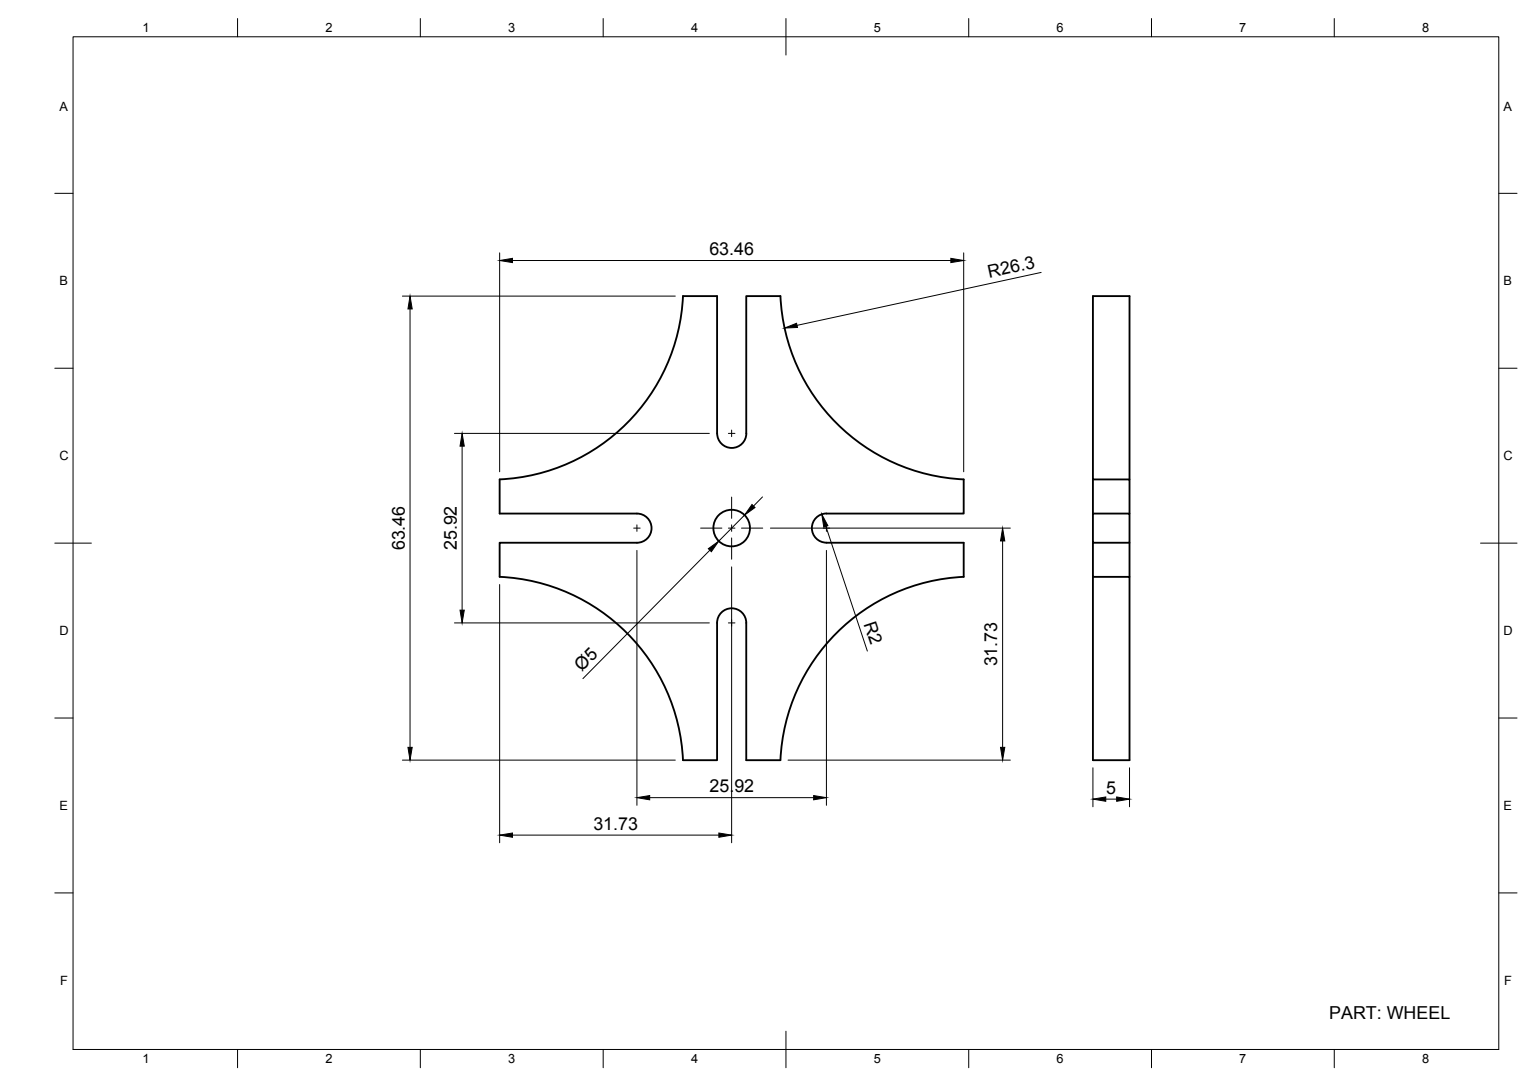
ISO-10303-21;
HEADER;
/* Generated by software containing ST-Developer
 * from STEP Tools, Inc. (www.steptools.com) 
 */

FILE_DESCRIPTION(
/* description */ (''),
/* implementation_level */ '2;1');

FILE_NAME(
/* name */ 'Wheel.step',
/* time_stamp */ '2026-09-20T21:52:48+06:00',
/* author */ (''),
/* organization */ (''),
/* preprocessor_version */ 'ST-DEVELOPER v20.2',
/* originating_system */ 'Autodesk Translation Framework v15.15.0.0',
/* authorisation */ '');

FILE_SCHEMA (('AUTOMOTIVE_DESIGN { 1 0 10303 214 3 1 1 }'));
ENDSEC;

DATA;
#10=MECHANICAL_DESIGN_GEOMETRIC_PRESENTATION_REPRESENTATION('',(#59),#2203);
#43=SHAPE_REPRESENTATION_RELATIONSHIP('SRR','None',#2235,#51);
#51=ADVANCED_BREP_SHAPE_REPRESENTATION('',(#67),#2195);
#59=STYLED_ITEM('',(#2284),#67);
#67=MANIFOLD_SOLID_BREP('Wheel',#1226);
#75=FACE_BOUND('',#256,.T.);
#76=FACE_BOUND('',#258,.T.);
#89=CIRCLE('',#1327,2.);
#90=CIRCLE('',#1328,2.);
#91=CIRCLE('',#1334,2.);
#92=CIRCLE('',#1335,2.);
#93=CIRCLE('',#1339,26.3);
#94=CIRCLE('',#1340,26.3);
#95=CIRCLE('',#1344,2.);
#96=CIRCLE('',#1345,2.);
#97=CIRCLE('',#1349,26.3);
#98=CIRCLE('',#1350,26.3);
#99=CIRCLE('',#1354,2.);
#100=CIRCLE('',#1355,2.);
#101=CIRCLE('',#1359,26.3);
#102=CIRCLE('',#1360,26.3);
#103=CIRCLE('',#1362,2.5);
#104=CIRCLE('',#1363,2.5);
#105=CIRCLE('',#1365,26.3);
#106=CIRCLE('',#1366,26.3);
#137=CYLINDRICAL_SURFACE('',#1326,2.);
#138=CYLINDRICAL_SURFACE('',#1333,2.);
#139=CYLINDRICAL_SURFACE('',#1338,26.3);
#140=CYLINDRICAL_SURFACE('',#1343,2.);
#141=CYLINDRICAL_SURFACE('',#1348,26.3);
#142=CYLINDRICAL_SURFACE('',#1353,2.);
#143=CYLINDRICAL_SURFACE('',#1358,26.3);
#144=CYLINDRICAL_SURFACE('',#1361,2.5);
#145=CYLINDRICAL_SURFACE('',#1364,26.3);
#161=FACE_OUTER_BOUND('',#230,.T.);
#162=FACE_OUTER_BOUND('',#231,.T.);
#163=FACE_OUTER_BOUND('',#232,.T.);
#164=FACE_OUTER_BOUND('',#233,.T.);
#165=FACE_OUTER_BOUND('',#234,.T.);
#166=FACE_OUTER_BOUND('',#235,.T.);
#167=FACE_OUTER_BOUND('',#236,.T.);
#168=FACE_OUTER_BOUND('',#237,.T.);
#169=FACE_OUTER_BOUND('',#238,.T.);
#170=FACE_OUTER_BOUND('',#239,.T.);
#171=FACE_OUTER_BOUND('',#240,.T.);
#172=FACE_OUTER_BOUND('',#241,.T.);
#173=FACE_OUTER_BOUND('',#242,.T.);
#174=FACE_OUTER_BOUND('',#243,.T.);
#175=FACE_OUTER_BOUND('',#244,.T.);
#176=FACE_OUTER_BOUND('',#245,.T.);
#177=FACE_OUTER_BOUND('',#246,.T.);
#178=FACE_OUTER_BOUND('',#247,.T.);
#179=FACE_OUTER_BOUND('',#248,.T.);
#180=FACE_OUTER_BOUND('',#249,.T.);
#181=FACE_OUTER_BOUND('',#250,.T.);
#182=FACE_OUTER_BOUND('',#251,.T.);
#183=FACE_OUTER_BOUND('',#252,.T.);
#184=FACE_OUTER_BOUND('',#253,.T.);
#185=FACE_OUTER_BOUND('',#254,.T.);
#186=FACE_OUTER_BOUND('',#255,.T.);
#187=FACE_OUTER_BOUND('',#257,.T.);
#230=EDGE_LOOP('',(#796,#797,#798,#799));
#231=EDGE_LOOP('',(#800,#801,#802,#803));
#232=EDGE_LOOP('',(#804,#805,#806,#807));
#233=EDGE_LOOP('',(#808,#809,#810,#811));
#234=EDGE_LOOP('',(#812,#813,#814,#815));
#235=EDGE_LOOP('',(#816,#817,#818,#819));
#236=EDGE_LOOP('',(#820,#821,#822,#823));
#237=EDGE_LOOP('',(#824,#825,#826,#827));
#238=EDGE_LOOP('',(#828,#829,#830,#831));
#239=EDGE_LOOP('',(#832,#833,#834,#835));
#240=EDGE_LOOP('',(#836,#837,#838,#839));
#241=EDGE_LOOP('',(#840,#841,#842,#843));
#242=EDGE_LOOP('',(#844,#845,#846,#847));
#243=EDGE_LOOP('',(#848,#849,#850,#851));
#244=EDGE_LOOP('',(#852,#853,#854,#855));
#245=EDGE_LOOP('',(#856,#857,#858,#859));
#246=EDGE_LOOP('',(#860,#861,#862,#863));
#247=EDGE_LOOP('',(#864,#865,#866,#867));
#248=EDGE_LOOP('',(#868,#869,#870,#871));
#249=EDGE_LOOP('',(#872,#873,#874,#875));
#250=EDGE_LOOP('',(#876,#877,#878,#879));
#251=EDGE_LOOP('',(#880,#881,#882,#883));
#252=EDGE_LOOP('',(#884,#885,#886,#887));
#253=EDGE_LOOP('',(#888,#889,#890,#891));
#254=EDGE_LOOP('',(#892,#893,#894,#895));
#255=EDGE_LOOP('',(#896,#897,#898,#899,#900,#901,#902,#903,#904,#905,#906,
#907,#908,#909,#910,#911,#912,#913,#914,#915,#916,#917,#918,#919));
#256=EDGE_LOOP('',(#920));
#257=EDGE_LOOP('',(#921,#922,#923,#924,#925,#926,#927,#928,#929,#930,#931,
#932,#933,#934,#935,#936,#937,#938,#939,#940,#941,#942,#943,#944));
#258=EDGE_LOOP('',(#945));
#313=LINE('',#1840,#423);
#314=LINE('',#1842,#424);
#315=LINE('',#1844,#425);
#316=LINE('',#1845,#426);
#317=LINE('',#1851,#427);
#318=LINE('',#1854,#428);
#319=LINE('',#1856,#429);
#320=LINE('',#1857,#430);
#321=LINE('',#1860,#431);
#322=LINE('',#1862,#432);
#323=LINE('',#1863,#433);
#324=LINE('',#1866,#434);
#325=LINE('',#1868,#435);
#326=LINE('',#1869,#436);
#327=LINE('',#1873,#437);
#328=LINE('',#1875,#438);
#329=LINE('',#1877,#439);
#330=LINE('',#1878,#440);
#331=LINE('',#1883,#441);
#332=LINE('',#1887,#442);
#333=LINE('',#1889,#443);
#334=LINE('',#1890,#444);
#335=LINE('',#1893,#445);
#336=LINE('',#1895,#446);
#337=LINE('',#1896,#447);
#338=LINE('',#1902,#448);
#339=LINE('',#1904,#449);
#340=LINE('',#1905,#450);
#341=LINE('',#1909,#451);
#342=LINE('',#1911,#452);
#343=LINE('',#1913,#453);
#344=LINE('',#1914,#454);
#345=LINE('',#1919,#455);
#346=LINE('',#1923,#456);
#347=LINE('',#1925,#457);
#348=LINE('',#1926,#458);
#349=LINE('',#1929,#459);
#350=LINE('',#1931,#460);
#351=LINE('',#1932,#461);
#352=LINE('',#1937,#462);
#353=LINE('',#1940,#463);
#354=LINE('',#1941,#464);
#355=LINE('',#1945,#465);
#356=LINE('',#1947,#466);
#357=LINE('',#1949,#467);
#358=LINE('',#1950,#468);
#359=LINE('',#1956,#469);
#360=LINE('',#1959,#470);
#361=LINE('',#1961,#471);
#362=LINE('',#1962,#472);
#363=LINE('',#1965,#473);
#364=LINE('',#1967,#474);
#365=LINE('',#1968,#475);
#366=LINE('',#1976,#476);
#367=LINE('',#1983,#477);
#368=LINE('',#1985,#478);
#369=LINE('',#1986,#479);
#423=VECTOR('',#1463,10.);
#424=VECTOR('',#1464,10.);
#425=VECTOR('',#1465,10.);
#426=VECTOR('',#1466,10.);
#427=VECTOR('',#1473,10.);
#428=VECTOR('',#1476,10.);
#429=VECTOR('',#1477,10.);
#430=VECTOR('',#1478,10.);
#431=VECTOR('',#1481,10.);
#432=VECTOR('',#1482,10.);
#433=VECTOR('',#1483,10.);
#434=VECTOR('',#1486,10.);
#435=VECTOR('',#1487,10.);
#436=VECTOR('',#1488,10.);
#437=VECTOR('',#1491,10.);
#438=VECTOR('',#1492,10.);
#439=VECTOR('',#1493,10.);
#440=VECTOR('',#1494,10.);
#441=VECTOR('',#1499,10.);
#442=VECTOR('',#1504,10.);
#443=VECTOR('',#1505,10.);
#444=VECTOR('',#1506,10.);
#445=VECTOR('',#1509,10.);
#446=VECTOR('',#1510,10.);
#447=VECTOR('',#1511,10.);
#448=VECTOR('',#1520,10.);
#449=VECTOR('',#1521,10.);
#450=VECTOR('',#1522,10.);
#451=VECTOR('',#1525,10.);
#452=VECTOR('',#1526,10.);
#453=VECTOR('',#1527,10.);
#454=VECTOR('',#1528,10.);
#455=VECTOR('',#1533,10.);
#456=VECTOR('',#1538,10.);
#457=VECTOR('',#1539,10.);
#458=VECTOR('',#1540,10.);
#459=VECTOR('',#1543,10.);
#460=VECTOR('',#1544,10.);
#461=VECTOR('',#1545,10.);
#462=VECTOR('',#1550,10.);
#463=VECTOR('',#1555,10.);
#464=VECTOR('',#1556,10.);
#465=VECTOR('',#1559,10.);
#466=VECTOR('',#1560,10.);
#467=VECTOR('',#1561,10.);
#468=VECTOR('',#1562,10.);
#469=VECTOR('',#1569,10.);
#470=VECTOR('',#1572,10.);
#471=VECTOR('',#1573,10.);
#472=VECTOR('',#1574,10.);
#473=VECTOR('',#1577,10.);
#474=VECTOR('',#1578,10.);
#475=VECTOR('',#1579,10.);
#476=VECTOR('',#1590,2.5);
#477=VECTOR('',#1599,10.);
#478=VECTOR('',#1602,10.);
#479=VECTOR('',#1603,10.);
#533=VERTEX_POINT('',#1838);
#534=VERTEX_POINT('',#1839);
#535=VERTEX_POINT('',#1841);
#536=VERTEX_POINT('',#1843);
#537=VERTEX_POINT('',#1847);
#538=VERTEX_POINT('',#1849);
#539=VERTEX_POINT('',#1853);
#540=VERTEX_POINT('',#1855);
#541=VERTEX_POINT('',#1859);
#542=VERTEX_POINT('',#1861);
#543=VERTEX_POINT('',#1865);
#544=VERTEX_POINT('',#1867);
#545=VERTEX_POINT('',#1871);
#546=VERTEX_POINT('',#1872);
#547=VERTEX_POINT('',#1874);
#548=VERTEX_POINT('',#1876);
#549=VERTEX_POINT('',#1880);
#550=VERTEX_POINT('',#1882);
#551=VERTEX_POINT('',#1886);
#552=VERTEX_POINT('',#1888);
#553=VERTEX_POINT('',#1892);
#554=VERTEX_POINT('',#1894);
#555=VERTEX_POINT('',#1901);
#556=VERTEX_POINT('',#1903);
#557=VERTEX_POINT('',#1907);
#558=VERTEX_POINT('',#1908);
#559=VERTEX_POINT('',#1910);
#560=VERTEX_POINT('',#1912);
#561=VERTEX_POINT('',#1916);
#562=VERTEX_POINT('',#1918);
#563=VERTEX_POINT('',#1922);
#564=VERTEX_POINT('',#1924);
#565=VERTEX_POINT('',#1928);
#566=VERTEX_POINT('',#1930);
#567=VERTEX_POINT('',#1934);
#568=VERTEX_POINT('',#1936);
#569=VERTEX_POINT('',#1943);
#570=VERTEX_POINT('',#1944);
#571=VERTEX_POINT('',#1946);
#572=VERTEX_POINT('',#1948);
#573=VERTEX_POINT('',#1952);
#574=VERTEX_POINT('',#1954);
#575=VERTEX_POINT('',#1958);
#576=VERTEX_POINT('',#1960);
#577=VERTEX_POINT('',#1964);
#578=VERTEX_POINT('',#1966);
#579=VERTEX_POINT('',#1973);
#580=VERTEX_POINT('',#1975);
#581=VERTEX_POINT('',#1979);
#582=VERTEX_POINT('',#1981);
#638=EDGE_CURVE('',#533,#534,#313,.T.);
#639=EDGE_CURVE('',#534,#535,#314,.T.);
#640=EDGE_CURVE('',#536,#535,#315,.T.);
#641=EDGE_CURVE('',#533,#536,#316,.T.);
#642=EDGE_CURVE('',#537,#533,#89,.T.);
#643=EDGE_CURVE('',#538,#536,#90,.T.);
#644=EDGE_CURVE('',#537,#538,#317,.T.);
#645=EDGE_CURVE('',#539,#537,#318,.T.);
#646=EDGE_CURVE('',#540,#538,#319,.T.);
#647=EDGE_CURVE('',#539,#540,#320,.T.);
#648=EDGE_CURVE('',#539,#541,#321,.T.);
#649=EDGE_CURVE('',#542,#540,#322,.T.);
#650=EDGE_CURVE('',#541,#542,#323,.T.);
#651=EDGE_CURVE('',#543,#534,#324,.T.);
#652=EDGE_CURVE('',#543,#544,#325,.T.);
#653=EDGE_CURVE('',#535,#544,#326,.T.);
#654=EDGE_CURVE('',#545,#546,#327,.T.);
#655=EDGE_CURVE('',#545,#547,#328,.T.);
#656=EDGE_CURVE('',#547,#548,#329,.T.);
#657=EDGE_CURVE('',#546,#548,#330,.T.);
#658=EDGE_CURVE('',#549,#545,#91,.T.);
#659=EDGE_CURVE('',#549,#550,#331,.T.);
#660=EDGE_CURVE('',#550,#547,#92,.T.);
#661=EDGE_CURVE('',#551,#549,#332,.T.);
#662=EDGE_CURVE('',#551,#552,#333,.T.);
#663=EDGE_CURVE('',#552,#550,#334,.T.);
#664=EDGE_CURVE('',#551,#553,#335,.T.);
#665=EDGE_CURVE('',#553,#554,#336,.T.);
#666=EDGE_CURVE('',#554,#552,#337,.T.);
#667=EDGE_CURVE('',#541,#553,#93,.T.);
#668=EDGE_CURVE('',#554,#542,#94,.T.);
#669=EDGE_CURVE('',#555,#546,#338,.T.);
#670=EDGE_CURVE('',#548,#556,#339,.T.);
#671=EDGE_CURVE('',#555,#556,#340,.T.);
#672=EDGE_CURVE('',#557,#558,#341,.T.);
#673=EDGE_CURVE('',#557,#559,#342,.T.);
#674=EDGE_CURVE('',#559,#560,#343,.T.);
#675=EDGE_CURVE('',#558,#560,#344,.T.);
#676=EDGE_CURVE('',#561,#557,#95,.T.);
#677=EDGE_CURVE('',#561,#562,#345,.T.);
#678=EDGE_CURVE('',#562,#559,#96,.T.);
#679=EDGE_CURVE('',#563,#561,#346,.T.);
#680=EDGE_CURVE('',#563,#564,#347,.T.);
#681=EDGE_CURVE('',#564,#562,#348,.T.);
#682=EDGE_CURVE('',#563,#565,#349,.T.);
#683=EDGE_CURVE('',#565,#566,#350,.T.);
#684=EDGE_CURVE('',#566,#564,#351,.T.);
#685=EDGE_CURVE('',#543,#567,#97,.T.);
#686=EDGE_CURVE('',#567,#568,#352,.T.);
#687=EDGE_CURVE('',#544,#568,#98,.T.);
#688=EDGE_CURVE('',#567,#558,#353,.T.);
#689=EDGE_CURVE('',#560,#568,#354,.T.);
#690=EDGE_CURVE('',#569,#570,#355,.T.);
#691=EDGE_CURVE('',#570,#571,#356,.T.);
#692=EDGE_CURVE('',#572,#571,#357,.T.);
#693=EDGE_CURVE('',#569,#572,#358,.T.);
#694=EDGE_CURVE('',#573,#569,#99,.T.);
#695=EDGE_CURVE('',#574,#572,#100,.T.);
#696=EDGE_CURVE('',#573,#574,#359,.T.);
#697=EDGE_CURVE('',#575,#573,#360,.T.);
#698=EDGE_CURVE('',#576,#574,#361,.T.);
#699=EDGE_CURVE('',#575,#576,#362,.T.);
#700=EDGE_CURVE('',#575,#577,#363,.T.);
#701=EDGE_CURVE('',#578,#576,#364,.T.);
#702=EDGE_CURVE('',#577,#578,#365,.T.);
#703=EDGE_CURVE('',#565,#577,#101,.T.);
#704=EDGE_CURVE('',#578,#566,#102,.T.);
#705=EDGE_CURVE('',#579,#579,#103,.T.);
#706=EDGE_CURVE('',#579,#580,#366,.T.);
#707=EDGE_CURVE('',#580,#580,#104,.T.);
#708=EDGE_CURVE('',#581,#555,#105,.T.);
#709=EDGE_CURVE('',#582,#556,#106,.T.);
#710=EDGE_CURVE('',#581,#582,#367,.T.);
#711=EDGE_CURVE('',#581,#570,#368,.T.);
#712=EDGE_CURVE('',#571,#582,#369,.T.);
#796=ORIENTED_EDGE('',*,*,#638,.T.);
#797=ORIENTED_EDGE('',*,*,#639,.T.);
#798=ORIENTED_EDGE('',*,*,#640,.F.);
#799=ORIENTED_EDGE('',*,*,#641,.F.);
#800=ORIENTED_EDGE('',*,*,#642,.T.);
#801=ORIENTED_EDGE('',*,*,#641,.T.);
#802=ORIENTED_EDGE('',*,*,#643,.F.);
#803=ORIENTED_EDGE('',*,*,#644,.F.);
#804=ORIENTED_EDGE('',*,*,#645,.T.);
#805=ORIENTED_EDGE('',*,*,#644,.T.);
#806=ORIENTED_EDGE('',*,*,#646,.F.);
#807=ORIENTED_EDGE('',*,*,#647,.F.);
#808=ORIENTED_EDGE('',*,*,#648,.F.);
#809=ORIENTED_EDGE('',*,*,#647,.T.);
#810=ORIENTED_EDGE('',*,*,#649,.F.);
#811=ORIENTED_EDGE('',*,*,#650,.F.);
#812=ORIENTED_EDGE('',*,*,#651,.F.);
#813=ORIENTED_EDGE('',*,*,#652,.T.);
#814=ORIENTED_EDGE('',*,*,#653,.F.);
#815=ORIENTED_EDGE('',*,*,#639,.F.);
#816=ORIENTED_EDGE('',*,*,#654,.F.);
#817=ORIENTED_EDGE('',*,*,#655,.T.);
#818=ORIENTED_EDGE('',*,*,#656,.T.);
#819=ORIENTED_EDGE('',*,*,#657,.F.);
#820=ORIENTED_EDGE('',*,*,#658,.F.);
#821=ORIENTED_EDGE('',*,*,#659,.T.);
#822=ORIENTED_EDGE('',*,*,#660,.T.);
#823=ORIENTED_EDGE('',*,*,#655,.F.);
#824=ORIENTED_EDGE('',*,*,#661,.F.);
#825=ORIENTED_EDGE('',*,*,#662,.T.);
#826=ORIENTED_EDGE('',*,*,#663,.T.);
#827=ORIENTED_EDGE('',*,*,#659,.F.);
#828=ORIENTED_EDGE('',*,*,#664,.T.);
#829=ORIENTED_EDGE('',*,*,#665,.T.);
#830=ORIENTED_EDGE('',*,*,#666,.T.);
#831=ORIENTED_EDGE('',*,*,#662,.F.);
#832=ORIENTED_EDGE('',*,*,#667,.F.);
#833=ORIENTED_EDGE('',*,*,#650,.T.);
#834=ORIENTED_EDGE('',*,*,#668,.F.);
#835=ORIENTED_EDGE('',*,*,#665,.F.);
#836=ORIENTED_EDGE('',*,*,#669,.T.);
#837=ORIENTED_EDGE('',*,*,#657,.T.);
#838=ORIENTED_EDGE('',*,*,#670,.T.);
#839=ORIENTED_EDGE('',*,*,#671,.F.);
#840=ORIENTED_EDGE('',*,*,#672,.F.);
#841=ORIENTED_EDGE('',*,*,#673,.T.);
#842=ORIENTED_EDGE('',*,*,#674,.T.);
#843=ORIENTED_EDGE('',*,*,#675,.F.);
#844=ORIENTED_EDGE('',*,*,#676,.F.);
#845=ORIENTED_EDGE('',*,*,#677,.T.);
#846=ORIENTED_EDGE('',*,*,#678,.T.);
#847=ORIENTED_EDGE('',*,*,#673,.F.);
#848=ORIENTED_EDGE('',*,*,#679,.F.);
#849=ORIENTED_EDGE('',*,*,#680,.T.);
#850=ORIENTED_EDGE('',*,*,#681,.T.);
#851=ORIENTED_EDGE('',*,*,#677,.F.);
#852=ORIENTED_EDGE('',*,*,#682,.T.);
#853=ORIENTED_EDGE('',*,*,#683,.T.);
#854=ORIENTED_EDGE('',*,*,#684,.T.);
#855=ORIENTED_EDGE('',*,*,#680,.F.);
#856=ORIENTED_EDGE('',*,*,#685,.T.);
#857=ORIENTED_EDGE('',*,*,#686,.T.);
#858=ORIENTED_EDGE('',*,*,#687,.F.);
#859=ORIENTED_EDGE('',*,*,#652,.F.);
#860=ORIENTED_EDGE('',*,*,#688,.T.);
#861=ORIENTED_EDGE('',*,*,#675,.T.);
#862=ORIENTED_EDGE('',*,*,#689,.T.);
#863=ORIENTED_EDGE('',*,*,#686,.F.);
#864=ORIENTED_EDGE('',*,*,#690,.T.);
#865=ORIENTED_EDGE('',*,*,#691,.T.);
#866=ORIENTED_EDGE('',*,*,#692,.F.);
#867=ORIENTED_EDGE('',*,*,#693,.F.);
#868=ORIENTED_EDGE('',*,*,#694,.T.);
#869=ORIENTED_EDGE('',*,*,#693,.T.);
#870=ORIENTED_EDGE('',*,*,#695,.F.);
#871=ORIENTED_EDGE('',*,*,#696,.F.);
#872=ORIENTED_EDGE('',*,*,#697,.T.);
#873=ORIENTED_EDGE('',*,*,#696,.T.);
#874=ORIENTED_EDGE('',*,*,#698,.F.);
#875=ORIENTED_EDGE('',*,*,#699,.F.);
#876=ORIENTED_EDGE('',*,*,#700,.F.);
#877=ORIENTED_EDGE('',*,*,#699,.T.);
#878=ORIENTED_EDGE('',*,*,#701,.F.);
#879=ORIENTED_EDGE('',*,*,#702,.F.);
#880=ORIENTED_EDGE('',*,*,#703,.T.);
#881=ORIENTED_EDGE('',*,*,#702,.T.);
#882=ORIENTED_EDGE('',*,*,#704,.T.);
#883=ORIENTED_EDGE('',*,*,#683,.F.);
#884=ORIENTED_EDGE('',*,*,#705,.T.);
#885=ORIENTED_EDGE('',*,*,#706,.T.);
#886=ORIENTED_EDGE('',*,*,#707,.T.);
#887=ORIENTED_EDGE('',*,*,#706,.F.);
#888=ORIENTED_EDGE('',*,*,#708,.T.);
#889=ORIENTED_EDGE('',*,*,#671,.T.);
#890=ORIENTED_EDGE('',*,*,#709,.F.);
#891=ORIENTED_EDGE('',*,*,#710,.F.);
#892=ORIENTED_EDGE('',*,*,#711,.F.);
#893=ORIENTED_EDGE('',*,*,#710,.T.);
#894=ORIENTED_EDGE('',*,*,#712,.F.);
#895=ORIENTED_EDGE('',*,*,#691,.F.);
#896=ORIENTED_EDGE('',*,*,#685,.F.);
#897=ORIENTED_EDGE('',*,*,#651,.T.);
#898=ORIENTED_EDGE('',*,*,#638,.F.);
#899=ORIENTED_EDGE('',*,*,#642,.F.);
#900=ORIENTED_EDGE('',*,*,#645,.F.);
#901=ORIENTED_EDGE('',*,*,#648,.T.);
#902=ORIENTED_EDGE('',*,*,#667,.T.);
#903=ORIENTED_EDGE('',*,*,#664,.F.);
#904=ORIENTED_EDGE('',*,*,#661,.T.);
#905=ORIENTED_EDGE('',*,*,#658,.T.);
#906=ORIENTED_EDGE('',*,*,#654,.T.);
#907=ORIENTED_EDGE('',*,*,#669,.F.);
#908=ORIENTED_EDGE('',*,*,#708,.F.);
#909=ORIENTED_EDGE('',*,*,#711,.T.);
#910=ORIENTED_EDGE('',*,*,#690,.F.);
#911=ORIENTED_EDGE('',*,*,#694,.F.);
#912=ORIENTED_EDGE('',*,*,#697,.F.);
#913=ORIENTED_EDGE('',*,*,#700,.T.);
#914=ORIENTED_EDGE('',*,*,#703,.F.);
#915=ORIENTED_EDGE('',*,*,#682,.F.);
#916=ORIENTED_EDGE('',*,*,#679,.T.);
#917=ORIENTED_EDGE('',*,*,#676,.T.);
#918=ORIENTED_EDGE('',*,*,#672,.T.);
#919=ORIENTED_EDGE('',*,*,#688,.F.);
#920=ORIENTED_EDGE('',*,*,#707,.F.);
#921=ORIENTED_EDGE('',*,*,#687,.T.);
#922=ORIENTED_EDGE('',*,*,#689,.F.);
#923=ORIENTED_EDGE('',*,*,#674,.F.);
#924=ORIENTED_EDGE('',*,*,#678,.F.);
#925=ORIENTED_EDGE('',*,*,#681,.F.);
#926=ORIENTED_EDGE('',*,*,#684,.F.);
#927=ORIENTED_EDGE('',*,*,#704,.F.);
#928=ORIENTED_EDGE('',*,*,#701,.T.);
#929=ORIENTED_EDGE('',*,*,#698,.T.);
#930=ORIENTED_EDGE('',*,*,#695,.T.);
#931=ORIENTED_EDGE('',*,*,#692,.T.);
#932=ORIENTED_EDGE('',*,*,#712,.T.);
#933=ORIENTED_EDGE('',*,*,#709,.T.);
#934=ORIENTED_EDGE('',*,*,#670,.F.);
#935=ORIENTED_EDGE('',*,*,#656,.F.);
#936=ORIENTED_EDGE('',*,*,#660,.F.);
#937=ORIENTED_EDGE('',*,*,#663,.F.);
#938=ORIENTED_EDGE('',*,*,#666,.F.);
#939=ORIENTED_EDGE('',*,*,#668,.T.);
#940=ORIENTED_EDGE('',*,*,#649,.T.);
#941=ORIENTED_EDGE('',*,*,#646,.T.);
#942=ORIENTED_EDGE('',*,*,#643,.T.);
#943=ORIENTED_EDGE('',*,*,#640,.T.);
#944=ORIENTED_EDGE('',*,*,#653,.T.);
#945=ORIENTED_EDGE('',*,*,#705,.F.);
#1112=PLANE('',#1325);
#1113=PLANE('',#1329);
#1114=PLANE('',#1330);
#1115=PLANE('',#1331);
#1116=PLANE('',#1332);
#1117=PLANE('',#1336);
#1118=PLANE('',#1337);
#1119=PLANE('',#1341);
#1120=PLANE('',#1342);
#1121=PLANE('',#1346);
#1122=PLANE('',#1347);
#1123=PLANE('',#1351);
#1124=PLANE('',#1352);
#1125=PLANE('',#1356);
#1126=PLANE('',#1357);
#1127=PLANE('',#1367);
#1128=PLANE('',#1368);
#1129=PLANE('',#1369);
#1157=ADVANCED_FACE('',(#161),#1112,.T.);
#1158=ADVANCED_FACE('',(#162),#137,.F.);
#1159=ADVANCED_FACE('',(#163),#1113,.T.);
#1160=ADVANCED_FACE('',(#164),#1114,.T.);
#1161=ADVANCED_FACE('',(#165),#1115,.T.);
#1162=ADVANCED_FACE('',(#166),#1116,.F.);
#1163=ADVANCED_FACE('',(#167),#138,.F.);
#1164=ADVANCED_FACE('',(#168),#1117,.F.);
#1165=ADVANCED_FACE('',(#169),#1118,.F.);
#1166=ADVANCED_FACE('',(#170),#139,.F.);
#1167=ADVANCED_FACE('',(#171),#1119,.F.);
#1168=ADVANCED_FACE('',(#172),#1120,.F.);
#1169=ADVANCED_FACE('',(#173),#140,.F.);
#1170=ADVANCED_FACE('',(#174),#1121,.F.);
#1171=ADVANCED_FACE('',(#175),#1122,.F.);
#1172=ADVANCED_FACE('',(#176),#141,.F.);
#1173=ADVANCED_FACE('',(#177),#1123,.F.);
#1174=ADVANCED_FACE('',(#178),#1124,.T.);
#1175=ADVANCED_FACE('',(#179),#142,.F.);
#1176=ADVANCED_FACE('',(#180),#1125,.T.);
#1177=ADVANCED_FACE('',(#181),#1126,.T.);
#1178=ADVANCED_FACE('',(#182),#143,.F.);
#1179=ADVANCED_FACE('',(#183),#144,.F.);
#1180=ADVANCED_FACE('',(#184),#145,.F.);
#1181=ADVANCED_FACE('',(#185),#1127,.T.);
#1182=ADVANCED_FACE('',(#186,#75),#1128,.T.);
#1183=ADVANCED_FACE('',(#187,#76),#1129,.F.);
#1226=CLOSED_SHELL('',(#1157,#1158,#1159,#1160,#1161,#1162,#1163,#1164,
#1165,#1166,#1167,#1168,#1169,#1170,#1171,#1172,#1173,#1174,#1175,#1176,
#1177,#1178,#1179,#1180,#1181,#1182,#1183));
#1324=AXIS2_PLACEMENT_3D('',#1836,#1459,#1460);
#1325=AXIS2_PLACEMENT_3D('',#1837,#1461,#1462);
#1326=AXIS2_PLACEMENT_3D('',#1846,#1467,#1468);
#1327=AXIS2_PLACEMENT_3D('',#1848,#1469,#1470);
#1328=AXIS2_PLACEMENT_3D('',#1850,#1471,#1472);
#1329=AXIS2_PLACEMENT_3D('',#1852,#1474,#1475);
#1330=AXIS2_PLACEMENT_3D('',#1858,#1479,#1480);
#1331=AXIS2_PLACEMENT_3D('',#1864,#1484,#1485);
#1332=AXIS2_PLACEMENT_3D('',#1870,#1489,#1490);
#1333=AXIS2_PLACEMENT_3D('',#1879,#1495,#1496);
#1334=AXIS2_PLACEMENT_3D('',#1881,#1497,#1498);
#1335=AXIS2_PLACEMENT_3D('',#1884,#1500,#1501);
#1336=AXIS2_PLACEMENT_3D('',#1885,#1502,#1503);
#1337=AXIS2_PLACEMENT_3D('',#1891,#1507,#1508);
#1338=AXIS2_PLACEMENT_3D('',#1897,#1512,#1513);
#1339=AXIS2_PLACEMENT_3D('',#1898,#1514,#1515);
#1340=AXIS2_PLACEMENT_3D('',#1899,#1516,#1517);
#1341=AXIS2_PLACEMENT_3D('',#1900,#1518,#1519);
#1342=AXIS2_PLACEMENT_3D('',#1906,#1523,#1524);
#1343=AXIS2_PLACEMENT_3D('',#1915,#1529,#1530);
#1344=AXIS2_PLACEMENT_3D('',#1917,#1531,#1532);
#1345=AXIS2_PLACEMENT_3D('',#1920,#1534,#1535);
#1346=AXIS2_PLACEMENT_3D('',#1921,#1536,#1537);
#1347=AXIS2_PLACEMENT_3D('',#1927,#1541,#1542);
#1348=AXIS2_PLACEMENT_3D('',#1933,#1546,#1547);
#1349=AXIS2_PLACEMENT_3D('',#1935,#1548,#1549);
#1350=AXIS2_PLACEMENT_3D('',#1938,#1551,#1552);
#1351=AXIS2_PLACEMENT_3D('',#1939,#1553,#1554);
#1352=AXIS2_PLACEMENT_3D('',#1942,#1557,#1558);
#1353=AXIS2_PLACEMENT_3D('',#1951,#1563,#1564);
#1354=AXIS2_PLACEMENT_3D('',#1953,#1565,#1566);
#1355=AXIS2_PLACEMENT_3D('',#1955,#1567,#1568);
#1356=AXIS2_PLACEMENT_3D('',#1957,#1570,#1571);
#1357=AXIS2_PLACEMENT_3D('',#1963,#1575,#1576);
#1358=AXIS2_PLACEMENT_3D('',#1969,#1580,#1581);
#1359=AXIS2_PLACEMENT_3D('',#1970,#1582,#1583);
#1360=AXIS2_PLACEMENT_3D('',#1971,#1584,#1585);
#1361=AXIS2_PLACEMENT_3D('',#1972,#1586,#1587);
#1362=AXIS2_PLACEMENT_3D('',#1974,#1588,#1589);
#1363=AXIS2_PLACEMENT_3D('',#1977,#1591,#1592);
#1364=AXIS2_PLACEMENT_3D('',#1978,#1593,#1594);
#1365=AXIS2_PLACEMENT_3D('',#1980,#1595,#1596);
#1366=AXIS2_PLACEMENT_3D('',#1982,#1597,#1598);
#1367=AXIS2_PLACEMENT_3D('',#1984,#1600,#1601);
#1368=AXIS2_PLACEMENT_3D('',#1987,#1604,#1605);
#1369=AXIS2_PLACEMENT_3D('',#1988,#1606,#1607);
#1459=DIRECTION('axis',(0.,0.,1.));
#1460=DIRECTION('refdir',(1.,0.,0.));
#1461=DIRECTION('center_axis',(0.707106781186548,0.,-0.707106781186547));
#1462=DIRECTION('ref_axis',(0.707106781186547,0.,0.707106781186548));
#1463=DIRECTION('',(0.707106781186547,0.,0.707106781186548));
#1464=DIRECTION('',(0.,-1.,0.));
#1465=DIRECTION('',(0.707106781186547,0.,0.707106781186548));
#1466=DIRECTION('',(0.,-1.,0.));
#1467=DIRECTION('center_axis',(0.,-1.,0.));
#1468=DIRECTION('ref_axis',(0.707106781186549,0.,-0.707106781186546));
#1469=DIRECTION('center_axis',(0.,1.,0.));
#1470=DIRECTION('ref_axis',(0.707106781186549,0.,-0.707106781186546));
#1471=DIRECTION('center_axis',(0.,1.,0.));
#1472=DIRECTION('ref_axis',(0.707106781186549,0.,-0.707106781186546));
#1473=DIRECTION('',(0.,-1.,0.));
#1474=DIRECTION('center_axis',(-0.707106781186548,0.,0.707106781186547));
#1475=DIRECTION('ref_axis',(-0.707106781186547,0.,-0.707106781186548));
#1476=DIRECTION('',(-0.707106781186547,0.,-0.707106781186548));
#1477=DIRECTION('',(-0.707106781186547,0.,-0.707106781186548));
#1478=DIRECTION('',(0.,-1.,0.));
#1479=DIRECTION('center_axis',(0.707106781186547,0.,0.707106781186548));
#1480=DIRECTION('ref_axis',(-0.707106781186548,0.,0.707106781186547));
#1481=DIRECTION('',(0.707106781186548,0.,-0.707106781186547));
#1482=DIRECTION('',(-0.707106781186548,0.,0.707106781186547));
#1483=DIRECTION('',(0.,-1.,0.));
#1484=DIRECTION('center_axis',(0.707106781186547,0.,0.707106781186548));
#1485=DIRECTION('ref_axis',(-0.707106781186548,0.,0.707106781186547));
#1486=DIRECTION('',(0.707106781186548,0.,-0.707106781186547));
#1487=DIRECTION('',(0.,-1.,0.));
#1488=DIRECTION('',(-0.707106781186548,0.,0.707106781186547));
#1489=DIRECTION('center_axis',(-0.707106781186548,0.,-0.707106781186547));
#1490=DIRECTION('ref_axis',(0.707106781186547,0.,-0.707106781186548));
#1491=DIRECTION('',(0.707106781186547,0.,-0.707106781186548));
#1492=DIRECTION('',(0.,-1.,0.));
#1493=DIRECTION('',(0.707106781186547,0.,-0.707106781186548));
#1494=DIRECTION('',(0.,-1.,0.));
#1495=DIRECTION('center_axis',(0.,1.,0.));
#1496=DIRECTION('ref_axis',(0.707106781186549,0.,0.707106781186546));
#1497=DIRECTION('center_axis',(0.,-1.,0.));
#1498=DIRECTION('ref_axis',(0.707106781186549,0.,0.707106781186546));
#1499=DIRECTION('',(0.,-1.,0.));
#1500=DIRECTION('center_axis',(0.,-1.,0.));
#1501=DIRECTION('ref_axis',(0.707106781186549,0.,0.707106781186546));
#1502=DIRECTION('center_axis',(0.707106781186548,0.,0.707106781186547));
#1503=DIRECTION('ref_axis',(-0.707106781186547,0.,0.707106781186548));
#1504=DIRECTION('',(-0.707106781186547,0.,0.707106781186548));
#1505=DIRECTION('',(0.,-1.,0.));
#1506=DIRECTION('',(-0.707106781186547,0.,0.707106781186548));
#1507=DIRECTION('center_axis',(-0.707106781186547,0.,0.707106781186548));
#1508=DIRECTION('ref_axis',(-0.707106781186548,0.,-0.707106781186547));
#1509=DIRECTION('',(0.707106781186548,0.,0.707106781186547));
#1510=DIRECTION('',(0.,-1.,0.));
#1511=DIRECTION('',(-0.707106781186548,0.,-0.707106781186547));
#1512=DIRECTION('center_axis',(0.,1.,0.));
#1513=DIRECTION('ref_axis',(-1.,0.,0.));
#1514=DIRECTION('center_axis',(0.,-1.,0.));
#1515=DIRECTION('ref_axis',(-1.,0.,0.));
#1516=DIRECTION('center_axis',(0.,1.,0.));
#1517=DIRECTION('ref_axis',(-1.,0.,0.));
#1518=DIRECTION('center_axis',(-0.707106781186547,0.,0.707106781186548));
#1519=DIRECTION('ref_axis',(-0.707106781186548,0.,-0.707106781186547));
#1520=DIRECTION('',(0.707106781186548,0.,0.707106781186547));
#1521=DIRECTION('',(-0.707106781186548,0.,-0.707106781186547));
#1522=DIRECTION('',(0.,-1.,0.));
#1523=DIRECTION('center_axis',(0.707106781186548,0.,0.707106781186547));
#1524=DIRECTION('ref_axis',(-0.707106781186547,0.,0.707106781186548));
#1525=DIRECTION('',(-0.707106781186547,0.,0.707106781186548));
#1526=DIRECTION('',(0.,-1.,0.));
#1527=DIRECTION('',(-0.707106781186547,0.,0.707106781186548));
#1528=DIRECTION('',(0.,-1.,0.));
#1529=DIRECTION('center_axis',(0.,1.,0.));
#1530=DIRECTION('ref_axis',(-0.707106781186549,0.,-0.707106781186546));
#1531=DIRECTION('center_axis',(0.,-1.,0.));
#1532=DIRECTION('ref_axis',(-0.707106781186549,0.,-0.707106781186546));
#1533=DIRECTION('',(0.,-1.,0.));
#1534=DIRECTION('center_axis',(0.,-1.,0.));
#1535=DIRECTION('ref_axis',(-0.707106781186549,0.,-0.707106781186546));
#1536=DIRECTION('center_axis',(-0.707106781186548,0.,-0.707106781186547));
#1537=DIRECTION('ref_axis',(0.707106781186547,0.,-0.707106781186548));
#1538=DIRECTION('',(0.707106781186547,0.,-0.707106781186548));
#1539=DIRECTION('',(0.,-1.,0.));
#1540=DIRECTION('',(0.707106781186547,0.,-0.707106781186548));
#1541=DIRECTION('center_axis',(0.707106781186547,0.,-0.707106781186548));
#1542=DIRECTION('ref_axis',(0.707106781186548,0.,0.707106781186547));
#1543=DIRECTION('',(-0.707106781186548,0.,-0.707106781186547));
#1544=DIRECTION('',(0.,-1.,0.));
#1545=DIRECTION('',(0.707106781186548,0.,0.707106781186547));
#1546=DIRECTION('center_axis',(0.,1.,0.));
#1547=DIRECTION('ref_axis',(1.,0.,0.));
#1548=DIRECTION('center_axis',(0.,1.,0.));
#1549=DIRECTION('ref_axis',(-1.,0.,0.));
#1550=DIRECTION('',(0.,-1.,0.));
#1551=DIRECTION('center_axis',(0.,1.,0.));
#1552=DIRECTION('ref_axis',(-1.,0.,0.));
#1553=DIRECTION('center_axis',(0.707106781186547,0.,-0.707106781186548));
#1554=DIRECTION('ref_axis',(0.707106781186548,0.,0.707106781186547));
#1555=DIRECTION('',(-0.707106781186548,0.,-0.707106781186547));
#1556=DIRECTION('',(0.707106781186548,0.,0.707106781186547));
#1557=DIRECTION('center_axis',(-0.707106781186548,0.,0.707106781186547));
#1558=DIRECTION('ref_axis',(-0.707106781186547,0.,-0.707106781186548));
#1559=DIRECTION('',(-0.707106781186547,0.,-0.707106781186548));
#1560=DIRECTION('',(0.,-1.,0.));
#1561=DIRECTION('',(-0.707106781186547,0.,-0.707106781186548));
#1562=DIRECTION('',(0.,-1.,0.));
#1563=DIRECTION('center_axis',(0.,-1.,0.));
#1564=DIRECTION('ref_axis',(-0.707106781186549,0.,0.707106781186546));
#1565=DIRECTION('center_axis',(0.,1.,0.));
#1566=DIRECTION('ref_axis',(-0.707106781186549,0.,0.707106781186546));
#1567=DIRECTION('center_axis',(0.,1.,0.));
#1568=DIRECTION('ref_axis',(-0.707106781186549,0.,0.707106781186546));
#1569=DIRECTION('',(0.,-1.,0.));
#1570=DIRECTION('center_axis',(0.707106781186548,0.,-0.707106781186547));
#1571=DIRECTION('ref_axis',(0.707106781186547,0.,0.707106781186548));
#1572=DIRECTION('',(0.707106781186547,0.,0.707106781186548));
#1573=DIRECTION('',(0.707106781186547,0.,0.707106781186548));
#1574=DIRECTION('',(0.,-1.,0.));
#1575=DIRECTION('center_axis',(-0.707106781186547,0.,-0.707106781186548));
#1576=DIRECTION('ref_axis',(0.707106781186548,0.,-0.707106781186547));
#1577=DIRECTION('',(-0.707106781186548,0.,0.707106781186547));
#1578=DIRECTION('',(0.707106781186548,0.,-0.707106781186547));
#1579=DIRECTION('',(0.,-1.,0.));
#1580=DIRECTION('center_axis',(0.,-1.,0.));
#1581=DIRECTION('ref_axis',(1.,0.,0.));
#1582=DIRECTION('center_axis',(0.,1.,0.));
#1583=DIRECTION('ref_axis',(1.,0.,0.));
#1584=DIRECTION('center_axis',(0.,-1.,0.));
#1585=DIRECTION('ref_axis',(1.,0.,0.));
#1586=DIRECTION('center_axis',(0.,-1.,0.));
#1587=DIRECTION('ref_axis',(1.,0.,0.));
#1588=DIRECTION('center_axis',(0.,-1.,0.));
#1589=DIRECTION('ref_axis',(-1.,0.,0.));
#1590=DIRECTION('',(0.,1.,0.));
#1591=DIRECTION('center_axis',(0.,1.,0.));
#1592=DIRECTION('ref_axis',(1.,0.,0.));
#1593=DIRECTION('center_axis',(0.,-1.,0.));
#1594=DIRECTION('ref_axis',(1.,0.,0.));
#1595=DIRECTION('center_axis',(0.,1.,0.));
#1596=DIRECTION('ref_axis',(1.,0.,0.));
#1597=DIRECTION('center_axis',(0.,1.,0.));
#1598=DIRECTION('ref_axis',(1.,0.,0.));
#1599=DIRECTION('',(0.,-1.,0.));
#1600=DIRECTION('center_axis',(-0.707106781186547,0.,-0.707106781186548));
#1601=DIRECTION('ref_axis',(0.707106781186548,0.,-0.707106781186547));
#1602=DIRECTION('',(-0.707106781186548,0.,0.707106781186547));
#1603=DIRECTION('',(0.707106781186548,0.,-0.707106781186547));
#1604=DIRECTION('center_axis',(0.,1.,0.));
#1605=DIRECTION('ref_axis',(1.,0.,0.));
#1606=DIRECTION('center_axis',(0.,1.,0.));
#1607=DIRECTION('ref_axis',(1.,0.,0.));
#1836=CARTESIAN_POINT('',(0.,0.,0.));
#1837=CARTESIAN_POINT('Origin',(7.75064923678082,0.,83.4550501631985));
#1838=CARTESIAN_POINT('',(7.7506492069785,0.,83.4550501333962));
#1839=CARTESIAN_POINT('',(21.0224285630747,0.,96.7268294894923));
#1840=CARTESIAN_POINT('',(7.75064923678082,0.,83.4550501631985));
#1841=CARTESIAN_POINT('',(21.0224285630747,-5.,96.7268294894923));
#1842=CARTESIAN_POINT('',(21.0224285630747,0.,96.7268294894923));
#1843=CARTESIAN_POINT('',(7.7506492069785,-5.,83.4550501333962));
#1844=CARTESIAN_POINT('',(7.75064923678082,-5.,83.4550501631985));
#1845=CARTESIAN_POINT('',(7.7506492069785,0.,83.4550501333962));
#1846=CARTESIAN_POINT('Origin',(9.16486279915392,0.,82.0408366008254));
#1847=CARTESIAN_POINT('',(10.579076361527,0.,80.6266230384523));
#1848=CARTESIAN_POINT('Origin',(9.16486279915392,0.,82.0408366008254));
#1849=CARTESIAN_POINT('',(10.579076361527,-5.,80.6266230384523));
#1850=CARTESIAN_POINT('Origin',(9.16486279915392,-5.,82.0408366008254));
#1851=CARTESIAN_POINT('',(10.579076361527,0.,80.6266230384523));
#1852=CARTESIAN_POINT('Origin',(23.8508556878209,0.,93.8984023647461));
#1853=CARTESIAN_POINT('',(23.8508556878209,0.,93.8984023647461));
#1854=CARTESIAN_POINT('',(25.6442326956396,0.,95.6917793725649));
#1855=CARTESIAN_POINT('',(23.8508556878209,-5.,93.8984023647461));
#1856=CARTESIAN_POINT('',(25.6442326956396,-5.,95.6917793725649));
#1857=CARTESIAN_POINT('',(23.8508556878209,0.,93.8984023647461));
#1858=CARTESIAN_POINT('Origin',(27.1472176868794,0.,90.6020403656876));
#1859=CARTESIAN_POINT('',(27.1472176868794,0.,90.6020403656876));
#1860=CARTESIAN_POINT('',(17.7260665640161,0.,100.023191488551));
#1861=CARTESIAN_POINT('',(27.1472176868794,-5.,90.6020403656876));
#1862=CARTESIAN_POINT('',(17.7260665640161,-5.,100.023191488551));
#1863=CARTESIAN_POINT('',(27.1472176868794,0.,90.6020403656876));
#1864=CARTESIAN_POINT('Origin',(21.0224285630747,0.,96.7268294894923));
#1865=CARTESIAN_POINT('',(17.7260665640161,0.,100.023191488551));
#1866=CARTESIAN_POINT('',(17.7260665640161,0.,100.023191488551));
#1867=CARTESIAN_POINT('',(17.7260665640161,-5.,100.023191488551));
#1868=CARTESIAN_POINT('',(17.7260665640161,0.,100.023191488551));
#1869=CARTESIAN_POINT('',(17.7260665640161,-5.,100.023191488551));
#1870=CARTESIAN_POINT('Origin',(7.75064923678082,0.,62.2968974401444));
#1871=CARTESIAN_POINT('',(7.7506492069785,0.,62.2968974699467));
#1872=CARTESIAN_POINT('',(21.0224285630747,0.,49.0251181138506));
#1873=CARTESIAN_POINT('',(7.75064923678082,0.,62.2968974401444));
#1874=CARTESIAN_POINT('',(7.7506492069785,-5.,62.2968974699467));
#1875=CARTESIAN_POINT('',(7.7506492069785,0.,62.2968974699467));
#1876=CARTESIAN_POINT('',(21.0224285630747,-5.,49.0251181138506));
#1877=CARTESIAN_POINT('',(7.75064923678082,-5.,62.2968974401444));
#1878=CARTESIAN_POINT('',(21.0224285630747,0.,49.0251181138506));
#1879=CARTESIAN_POINT('Origin',(9.16486279915392,0.,63.7111110025175));
#1880=CARTESIAN_POINT('',(10.579076361527,0.,65.1253245648906));
#1881=CARTESIAN_POINT('Origin',(9.16486279915392,0.,63.7111110025175));
#1882=CARTESIAN_POINT('',(10.579076361527,-5.,65.1253245648906));
#1883=CARTESIAN_POINT('',(10.579076361527,0.,65.1253245648906));
#1884=CARTESIAN_POINT('Origin',(9.16486279915392,-5.,63.7111110025175));
#1885=CARTESIAN_POINT('Origin',(23.8508556878209,0.,51.8535452385968));
#1886=CARTESIAN_POINT('',(23.8508556878209,0.,51.8535452385968));
#1887=CARTESIAN_POINT('',(25.6442326956396,0.,50.060168230778));
#1888=CARTESIAN_POINT('',(23.8508556878209,-5.,51.8535452385968));
#1889=CARTESIAN_POINT('',(23.8508556878209,0.,51.8535452385968));
#1890=CARTESIAN_POINT('',(25.6442326956396,-5.,50.060168230778));
#1891=CARTESIAN_POINT('Origin',(27.1472176868794,0.,55.1499072376553));
#1892=CARTESIAN_POINT('',(27.1472176868794,0.,55.1499072376553));
#1893=CARTESIAN_POINT('',(17.7260665640161,0.,45.728756114792));
#1894=CARTESIAN_POINT('',(27.1472176868794,-5.,55.1499072376553));
#1895=CARTESIAN_POINT('',(27.1472176868794,0.,55.1499072376553));
#1896=CARTESIAN_POINT('',(17.7260665640161,-5.,45.728756114792));
#1897=CARTESIAN_POINT('Origin',(46.5759738016714,0.,72.8759738016714));
#1898=CARTESIAN_POINT('Origin',(46.5759738016714,0.,72.8759738016714));
#1899=CARTESIAN_POINT('Origin',(46.5759738016714,-5.,72.8759738016714));
#1900=CARTESIAN_POINT('Origin',(21.0224285630747,0.,49.0251181138506));
#1901=CARTESIAN_POINT('',(17.7260665640161,0.,45.728756114792));
#1902=CARTESIAN_POINT('',(17.7260665640161,0.,45.728756114792));
#1903=CARTESIAN_POINT('',(17.7260665640161,-5.,45.728756114792));
#1904=CARTESIAN_POINT('',(17.7260665640161,-5.,45.728756114792));
#1905=CARTESIAN_POINT('',(17.7260665640161,0.,45.728756114792));
#1906=CARTESIAN_POINT('Origin',(-7.75064923678082,0.,83.4550501631985));
#1907=CARTESIAN_POINT('',(-7.7506492069785,0.,83.4550501333962));
#1908=CARTESIAN_POINT('',(-21.0224285630747,0.,96.7268294894923));
#1909=CARTESIAN_POINT('',(-7.75064923678082,0.,83.4550501631985));
#1910=CARTESIAN_POINT('',(-7.7506492069785,-5.,83.4550501333962));
#1911=CARTESIAN_POINT('',(-7.7506492069785,0.,83.4550501333962));
#1912=CARTESIAN_POINT('',(-21.0224285630747,-5.,96.7268294894923));
#1913=CARTESIAN_POINT('',(-7.75064923678082,-5.,83.4550501631985));
#1914=CARTESIAN_POINT('',(-21.0224285630747,0.,96.7268294894923));
#1915=CARTESIAN_POINT('Origin',(-9.16486279915392,0.,82.0408366008254));
#1916=CARTESIAN_POINT('',(-10.579076361527,0.,80.6266230384523));
#1917=CARTESIAN_POINT('Origin',(-9.16486279915392,0.,82.0408366008254));
#1918=CARTESIAN_POINT('',(-10.579076361527,-5.,80.6266230384523));
#1919=CARTESIAN_POINT('',(-10.579076361527,0.,80.6266230384523));
#1920=CARTESIAN_POINT('Origin',(-9.16486279915392,-5.,82.0408366008254));
#1921=CARTESIAN_POINT('Origin',(-23.8508556878209,0.,93.8984023647461));
#1922=CARTESIAN_POINT('',(-23.8508556878209,0.,93.8984023647461));
#1923=CARTESIAN_POINT('',(-25.6442326956396,0.,95.6917793725649));
#1924=CARTESIAN_POINT('',(-23.8508556878209,-5.,93.8984023647461));
#1925=CARTESIAN_POINT('',(-23.8508556878209,0.,93.8984023647461));
#1926=CARTESIAN_POINT('',(-25.6442326956396,-5.,95.6917793725649));
#1927=CARTESIAN_POINT('Origin',(-27.1472176868794,0.,90.6020403656876));
#1928=CARTESIAN_POINT('',(-27.1472176868794,0.,90.6020403656876));
#1929=CARTESIAN_POINT('',(-17.7260665640161,0.,100.023191488551));
#1930=CARTESIAN_POINT('',(-27.1472176868794,-5.,90.6020403656876));
#1931=CARTESIAN_POINT('',(-27.1472176868794,0.,90.6020403656876));
#1932=CARTESIAN_POINT('',(-17.7260665640161,-5.,100.023191488551));
#1933=CARTESIAN_POINT('Origin',(0.,0.,119.451947603343));
#1934=CARTESIAN_POINT('',(-17.7260665640161,0.,100.023191488551));
#1935=CARTESIAN_POINT('Origin',(1.53080849893419E-15,0.,119.451947603343));
#1936=CARTESIAN_POINT('',(-17.7260665640161,-5.,100.023191488551));
#1937=CARTESIAN_POINT('',(-17.7260665640161,0.,100.023191488551));
#1938=CARTESIAN_POINT('Origin',(1.53080849893419E-15,-5.,119.451947603343));
#1939=CARTESIAN_POINT('Origin',(-21.0224285630747,0.,96.7268294894923));
#1940=CARTESIAN_POINT('',(-17.7260665640161,0.,100.023191488551));
#1941=CARTESIAN_POINT('',(-17.7260665640161,-5.,100.023191488551));
#1942=CARTESIAN_POINT('Origin',(-7.75064923678082,0.,62.2968974401444));
#1943=CARTESIAN_POINT('',(-7.7506492069785,0.,62.2968974699467));
#1944=CARTESIAN_POINT('',(-21.0224285630747,0.,49.0251181138506));
#1945=CARTESIAN_POINT('',(-7.75064923678082,0.,62.2968974401444));
#1946=CARTESIAN_POINT('',(-21.0224285630747,-5.,49.0251181138506));
#1947=CARTESIAN_POINT('',(-21.0224285630747,0.,49.0251181138506));
#1948=CARTESIAN_POINT('',(-7.7506492069785,-5.,62.2968974699467));
#1949=CARTESIAN_POINT('',(-7.75064923678082,-5.,62.2968974401444));
#1950=CARTESIAN_POINT('',(-7.7506492069785,0.,62.2968974699467));
#1951=CARTESIAN_POINT('Origin',(-9.16486279915392,0.,63.7111110025175));
#1952=CARTESIAN_POINT('',(-10.579076361527,0.,65.1253245648906));
#1953=CARTESIAN_POINT('Origin',(-9.16486279915392,0.,63.7111110025175));
#1954=CARTESIAN_POINT('',(-10.579076361527,-5.,65.1253245648906));
#1955=CARTESIAN_POINT('Origin',(-9.16486279915392,-5.,63.7111110025175));
#1956=CARTESIAN_POINT('',(-10.579076361527,0.,65.1253245648906));
#1957=CARTESIAN_POINT('Origin',(-23.8508556878209,0.,51.8535452385968));
#1958=CARTESIAN_POINT('',(-23.8508556878209,0.,51.8535452385968));
#1959=CARTESIAN_POINT('',(-25.6442326956396,0.,50.060168230778));
#1960=CARTESIAN_POINT('',(-23.8508556878209,-5.,51.8535452385968));
#1961=CARTESIAN_POINT('',(-25.6442326956396,-5.,50.060168230778));
#1962=CARTESIAN_POINT('',(-23.8508556878209,0.,51.8535452385968));
#1963=CARTESIAN_POINT('Origin',(-27.1472176868794,0.,55.1499072376553));
#1964=CARTESIAN_POINT('',(-27.1472176868794,0.,55.1499072376553));
#1965=CARTESIAN_POINT('',(-17.7260665640161,0.,45.728756114792));
#1966=CARTESIAN_POINT('',(-27.1472176868794,-5.,55.1499072376553));
#1967=CARTESIAN_POINT('',(-17.7260665640161,-5.,45.728756114792));
#1968=CARTESIAN_POINT('',(-27.1472176868794,0.,55.1499072376553));
#1969=CARTESIAN_POINT('Origin',(-46.5759738016714,0.,72.8759738016714));
#1970=CARTESIAN_POINT('Origin',(-46.5759738016714,0.,72.8759738016714));
#1971=CARTESIAN_POINT('Origin',(-46.5759738016714,-5.,72.8759738016714));
#1972=CARTESIAN_POINT('Origin',(0.,0.,72.8759738016714));
#1973=CARTESIAN_POINT('',(-2.5,-5.,72.8759738016714));
#1974=CARTESIAN_POINT('Origin',(1.53080849893419E-15,-5.,72.8759738016714));
#1975=CARTESIAN_POINT('',(-2.5,0.,72.8759738016714));
#1976=CARTESIAN_POINT('',(-2.5,0.,72.8759738016714));
#1977=CARTESIAN_POINT('Origin',(0.,0.,72.8759738016714));
#1978=CARTESIAN_POINT('Origin',(0.,0.,26.3));
#1979=CARTESIAN_POINT('',(-17.7260665640161,0.,45.728756114792));
#1980=CARTESIAN_POINT('Origin',(0.,0.,26.3));
#1981=CARTESIAN_POINT('',(-17.7260665640161,-5.,45.728756114792));
#1982=CARTESIAN_POINT('Origin',(0.,-5.,26.3));
#1983=CARTESIAN_POINT('',(-17.7260665640161,0.,45.728756114792));
#1984=CARTESIAN_POINT('Origin',(-21.0224285630747,0.,49.0251181138506));
#1985=CARTESIAN_POINT('',(-17.7260665640161,0.,45.728756114792));
#1986=CARTESIAN_POINT('',(-17.7260665640161,-5.,45.728756114792));
#1987=CARTESIAN_POINT('Origin',(-13.5736088434397,0.,59.3023649582317));
#1988=CARTESIAN_POINT('Origin',(-13.5736088434397,-5.,59.3023649582317));
#2185=UNCERTAINTY_MEASURE_WITH_UNIT(LENGTH_MEASURE(0.01),#2204,
'DISTANCE_ACCURACY_VALUE',
'Maximum model space distance between geometric entities at asserted c
onnectivities');
#2193=UNCERTAINTY_MEASURE_WITH_UNIT(LENGTH_MEASURE(0.01),#2204,
'DISTANCE_ACCURACY_VALUE',
'Maximum model space distance between geometric entities at asserted c
onnectivities');
#2195=(
GEOMETRIC_REPRESENTATION_CONTEXT(3)
GLOBAL_UNCERTAINTY_ASSIGNED_CONTEXT((#2185))
GLOBAL_UNIT_ASSIGNED_CONTEXT((#2204,#2206,#2207))
REPRESENTATION_CONTEXT('','3D')
);
#2203=(
GEOMETRIC_REPRESENTATION_CONTEXT(3)
GLOBAL_UNCERTAINTY_ASSIGNED_CONTEXT((#2193))
GLOBAL_UNIT_ASSIGNED_CONTEXT((#2204,#2206,#2207))
REPRESENTATION_CONTEXT('','3D')
);
#2204=(
LENGTH_UNIT()
NAMED_UNIT(*)
SI_UNIT(.MILLI.,.METRE.)
);
#2206=(
NAMED_UNIT(*)
PLANE_ANGLE_UNIT()
SI_UNIT($,.RADIAN.)
);
#2207=(
NAMED_UNIT(*)
SI_UNIT($,.STERADIAN.)
SOLID_ANGLE_UNIT()
);
#2209=SHAPE_DEFINITION_REPRESENTATION(#2218,#2235);
#2218=PRODUCT_DEFINITION_SHAPE('',$,#2245);
#2235=SHAPE_REPRESENTATION('',(#1324),#2195);
#2243=PRODUCT_DEFINITION_CONTEXT('part definition',#2272,'design');
#2245=PRODUCT_DEFINITION('Wheel','Wheel',#2254,#2243);
#2254=PRODUCT_DEFINITION_FORMATION('',$,#2275);
#2272=APPLICATION_CONTEXT(
'Core Data for Automotive Mechanical Design Process');
#2273=PRODUCT_CONTEXT('part definition',#2272,'mechanical');
#2275=PRODUCT('Wheel','Wheel',$,(#2273));
#2284=PRESENTATION_STYLE_ASSIGNMENT((#2288));
#2288=SURFACE_STYLE_USAGE(.BOTH.,#2292);
#2292=SURFACE_SIDE_STYLE('',(#2296));
#2296=SURFACE_STYLE_FILL_AREA(#2300);
#2300=FILL_AREA_STYLE('Surface - Matte',(#2304));
#2304=FILL_AREA_STYLE_COLOUR('Surface - Matte',#2308);
#2308=COLOUR_RGB('Surface - Matte', 0.09019608, 0.27058824, 0.51372549);
ENDSEC;
END-ISO-10303-21;
